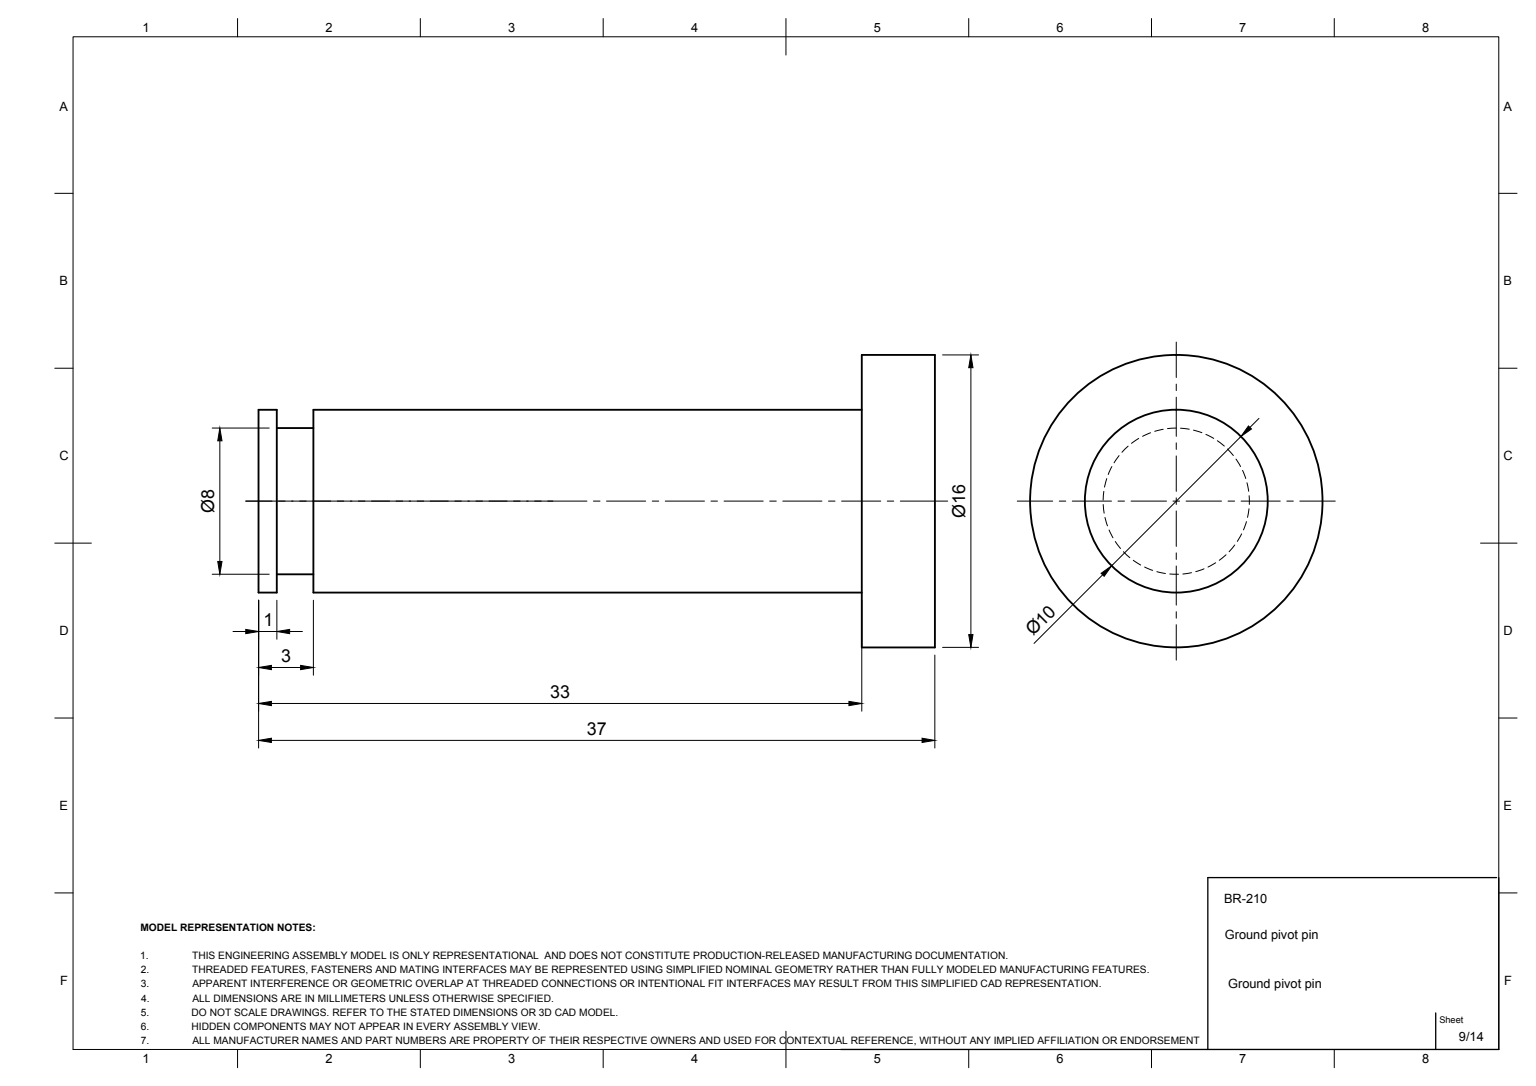
ISO-10303-21;
HEADER;
/* Generated by software containing ST-Developer
 * from STEP Tools, Inc. (www.steptools.com) 
 */

FILE_DESCRIPTION(
/* description */ ('Independent 1:2 reduction pantograph. 120 mm parallelogram sides; fix
ed fulcrum on the extension of a 240 mm link. Drawing point halfway al
ong its link, so its XY displacement is one half of the tracing point.
 Replaceable pivot bushes and retained pins. Calibration and productio
n accuracy unassigned.'),
/* implementation_level */ '2;1');

FILE_NAME(
/* name */ 'Ground pivot pin.step',
/* time_stamp */ '2026-11-07T22:11:57-08:00',
/* author */ (''),
/* organization */ (''),
/* preprocessor_version */ 'ST-DEVELOPER v20.2',
/* originating_system */ 'Autodesk Translation Framework v15.17.0.0',
/* authorisation */ '');

FILE_SCHEMA (('AUTOMOTIVE_DESIGN { 1 0 10303 214 3 1 1 }'));
ENDSEC;

DATA;
#10=MECHANICAL_DESIGN_GEOMETRIC_PRESENTATION_REPRESENTATION('',(#190),#2926);
#164=SHAPE_REPRESENTATION_RELATIONSHIP('SRR','None',#3001,#177);
#177=ADVANCED_BREP_SHAPE_REPRESENTATION('',(#203),#2917);
#190=STYLED_ITEM('',(#3075),#203);
#203=MANIFOLD_SOLID_BREP('Body1',#1545);
#236=FACE_BOUND('',#456,.T.);
#237=FACE_BOUND('',#458,.T.);
#238=FACE_BOUND('',#461,.T.);
#274=PLANE('',#1774);
#275=PLANE('',#1776);
#276=PLANE('',#1780);
#277=PLANE('',#1785);
#278=PLANE('',#1787);
#338=FACE_OUTER_BOUND('',#454,.T.);
#339=FACE_OUTER_BOUND('',#455,.T.);
#340=FACE_OUTER_BOUND('',#457,.T.);
#341=FACE_OUTER_BOUND('',#459,.T.);
#342=FACE_OUTER_BOUND('',#460,.T.);
#343=FACE_OUTER_BOUND('',#462,.T.);
#344=FACE_OUTER_BOUND('',#463,.T.);
#345=FACE_OUTER_BOUND('',#464,.T.);
#346=FACE_OUTER_BOUND('',#465,.T.);
#454=EDGE_LOOP('',(#1217,#1218,#1219,#1220));
#455=EDGE_LOOP('',(#1221));
#456=EDGE_LOOP('',(#1222));
#457=EDGE_LOOP('',(#1223));
#458=EDGE_LOOP('',(#1224));
#459=EDGE_LOOP('',(#1225,#1226,#1227,#1228));
#460=EDGE_LOOP('',(#1229));
#461=EDGE_LOOP('',(#1230));
#462=EDGE_LOOP('',(#1231,#1232,#1233,#1234));
#463=EDGE_LOOP('',(#1235));
#464=EDGE_LOOP('',(#1236,#1237,#1238,#1239));
#465=EDGE_LOOP('',(#1240));
#576=LINE('',#2640,#657);
#577=LINE('',#2651,#658);
#578=LINE('',#2659,#659);
#579=LINE('',#2663,#660);
#657=VECTOR('',#2120,4.);
#658=VECTOR('',#2135,5.);
#659=VECTOR('',#2144,8.);
#660=VECTOR('',#2151,5.);
#731=CIRCLE('',#1772,4.);
#732=CIRCLE('',#1773,4.);
#733=CIRCLE('',#1775,5.);
#734=CIRCLE('',#1777,5.);
#735=CIRCLE('',#1779,5.);
#736=CIRCLE('',#1781,8.);
#737=CIRCLE('',#1782,5.);
#738=CIRCLE('',#1784,8.);
#835=VERTEX_POINT('',#2637);
#836=VERTEX_POINT('',#2639);
#837=VERTEX_POINT('',#2643);
#838=VERTEX_POINT('',#2646);
#839=VERTEX_POINT('',#2649);
#840=VERTEX_POINT('',#2653);
#841=VERTEX_POINT('',#2655);
#842=VERTEX_POINT('',#2658);
#973=EDGE_CURVE('',#835,#835,#731,.T.);
#974=EDGE_CURVE('',#835,#836,#576,.T.);
#975=EDGE_CURVE('',#836,#836,#732,.T.);
#976=EDGE_CURVE('',#837,#837,#733,.T.);
#977=EDGE_CURVE('',#838,#838,#734,.T.);
#978=EDGE_CURVE('',#839,#839,#735,.T.);
#979=EDGE_CURVE('',#839,#838,#577,.T.);
#980=EDGE_CURVE('',#840,#840,#736,.T.);
#981=EDGE_CURVE('',#841,#841,#737,.T.);
#982=EDGE_CURVE('',#840,#842,#578,.T.);
#983=EDGE_CURVE('',#842,#842,#738,.T.);
#984=EDGE_CURVE('',#837,#841,#579,.T.);
#1217=ORIENTED_EDGE('',*,*,#973,.T.);
#1218=ORIENTED_EDGE('',*,*,#974,.T.);
#1219=ORIENTED_EDGE('',*,*,#975,.F.);
#1220=ORIENTED_EDGE('',*,*,#974,.F.);
#1221=ORIENTED_EDGE('',*,*,#976,.F.);
#1222=ORIENTED_EDGE('',*,*,#973,.F.);
#1223=ORIENTED_EDGE('',*,*,#977,.F.);
#1224=ORIENTED_EDGE('',*,*,#975,.T.);
#1225=ORIENTED_EDGE('',*,*,#978,.F.);
#1226=ORIENTED_EDGE('',*,*,#979,.T.);
#1227=ORIENTED_EDGE('',*,*,#977,.T.);
#1228=ORIENTED_EDGE('',*,*,#979,.F.);
#1229=ORIENTED_EDGE('',*,*,#980,.T.);
#1230=ORIENTED_EDGE('',*,*,#981,.F.);
#1231=ORIENTED_EDGE('',*,*,#980,.F.);
#1232=ORIENTED_EDGE('',*,*,#982,.T.);
#1233=ORIENTED_EDGE('',*,*,#983,.T.);
#1234=ORIENTED_EDGE('',*,*,#982,.F.);
#1235=ORIENTED_EDGE('',*,*,#983,.F.);
#1236=ORIENTED_EDGE('',*,*,#976,.T.);
#1237=ORIENTED_EDGE('',*,*,#984,.T.);
#1238=ORIENTED_EDGE('',*,*,#981,.T.);
#1239=ORIENTED_EDGE('',*,*,#984,.F.);
#1240=ORIENTED_EDGE('',*,*,#978,.T.);
#1422=CYLINDRICAL_SURFACE('',#1771,4.);
#1423=CYLINDRICAL_SURFACE('',#1778,5.);
#1424=CYLINDRICAL_SURFACE('',#1783,8.);
#1425=CYLINDRICAL_SURFACE('',#1786,5.);
#1482=ADVANCED_FACE('',(#338),#1422,.T.);
#1483=ADVANCED_FACE('',(#339,#236),#274,.F.);
#1484=ADVANCED_FACE('',(#340,#237),#275,.F.);
#1485=ADVANCED_FACE('',(#341),#1423,.T.);
#1486=ADVANCED_FACE('',(#342,#238),#276,.T.);
#1487=ADVANCED_FACE('',(#343),#1424,.T.);
#1488=ADVANCED_FACE('',(#344),#277,.F.);
#1489=ADVANCED_FACE('',(#345),#1425,.T.);
#1490=ADVANCED_FACE('',(#346),#278,.T.);
#1545=CLOSED_SHELL('',(#1482,#1483,#1484,#1485,#1486,#1487,#1488,#1489,
#1490));
#1770=AXIS2_PLACEMENT_3D('',#2635,#2114,#2115);
#1771=AXIS2_PLACEMENT_3D('',#2636,#2116,#2117);
#1772=AXIS2_PLACEMENT_3D('',#2638,#2118,#2119);
#1773=AXIS2_PLACEMENT_3D('',#2641,#2121,#2122);
#1774=AXIS2_PLACEMENT_3D('',#2642,#2123,#2124);
#1775=AXIS2_PLACEMENT_3D('',#2644,#2125,#2126);
#1776=AXIS2_PLACEMENT_3D('',#2645,#2127,#2128);
#1777=AXIS2_PLACEMENT_3D('',#2647,#2129,#2130);
#1778=AXIS2_PLACEMENT_3D('',#2648,#2131,#2132);
#1779=AXIS2_PLACEMENT_3D('',#2650,#2133,#2134);
#1780=AXIS2_PLACEMENT_3D('',#2652,#2136,#2137);
#1781=AXIS2_PLACEMENT_3D('',#2654,#2138,#2139);
#1782=AXIS2_PLACEMENT_3D('',#2656,#2140,#2141);
#1783=AXIS2_PLACEMENT_3D('',#2657,#2142,#2143);
#1784=AXIS2_PLACEMENT_3D('',#2660,#2145,#2146);
#1785=AXIS2_PLACEMENT_3D('',#2661,#2147,#2148);
#1786=AXIS2_PLACEMENT_3D('',#2662,#2149,#2150);
#1787=AXIS2_PLACEMENT_3D('',#2664,#2152,#2153);
#2114=DIRECTION('axis',(0.,0.,1.));
#2115=DIRECTION('refdir',(1.,0.,0.));
#2116=DIRECTION('center_axis',(0.,0.,1.));
#2117=DIRECTION('ref_axis',(1.,0.,0.));
#2118=DIRECTION('center_axis',(0.,0.,1.));
#2119=DIRECTION('ref_axis',(1.,0.,0.));
#2120=DIRECTION('',(0.,0.,1.));
#2121=DIRECTION('center_axis',(0.,0.,1.));
#2122=DIRECTION('ref_axis',(1.,0.,0.));
#2123=DIRECTION('center_axis',(0.,0.,-1.));
#2124=DIRECTION('ref_axis',(-1.,0.,0.));
#2125=DIRECTION('center_axis',(0.,0.,-1.));
#2126=DIRECTION('ref_axis',(1.,0.,0.));
#2127=DIRECTION('center_axis',(0.,0.,1.));
#2128=DIRECTION('ref_axis',(1.,0.,0.));
#2129=DIRECTION('center_axis',(0.,0.,1.));
#2130=DIRECTION('ref_axis',(1.,0.,0.));
#2131=DIRECTION('center_axis',(0.,0.,1.));
#2132=DIRECTION('ref_axis',(1.,0.,0.));
#2133=DIRECTION('center_axis',(0.,0.,1.));
#2134=DIRECTION('ref_axis',(1.,0.,0.));
#2135=DIRECTION('',(0.,0.,-1.));
#2136=DIRECTION('center_axis',(0.,0.,1.));
#2137=DIRECTION('ref_axis',(1.,0.,0.));
#2138=DIRECTION('center_axis',(0.,0.,1.));
#2139=DIRECTION('ref_axis',(1.,0.,0.));
#2140=DIRECTION('center_axis',(0.,0.,1.));
#2141=DIRECTION('ref_axis',(1.,0.,0.));
#2142=DIRECTION('center_axis',(0.,0.,1.));
#2143=DIRECTION('ref_axis',(1.,0.,0.));
#2144=DIRECTION('',(0.,0.,-1.));
#2145=DIRECTION('center_axis',(0.,0.,1.));
#2146=DIRECTION('ref_axis',(1.,0.,0.));
#2147=DIRECTION('center_axis',(0.,0.,1.));
#2148=DIRECTION('ref_axis',(1.,0.,0.));
#2149=DIRECTION('center_axis',(0.,0.,1.));
#2150=DIRECTION('ref_axis',(1.,0.,0.));
#2151=DIRECTION('',(0.,0.,-1.));
#2152=DIRECTION('center_axis',(0.,0.,1.));
#2153=DIRECTION('ref_axis',(1.,0.,0.));
#2635=CARTESIAN_POINT('',(0.,0.,0.));
#2636=CARTESIAN_POINT('Origin',(0.,0.,31.));
#2637=CARTESIAN_POINT('',(-4.,-4.89858719658941E-16,30.));
#2638=CARTESIAN_POINT('Origin',(0.,0.,30.));
#2639=CARTESIAN_POINT('',(-4.,-4.89858719658941E-16,32.));
#2640=CARTESIAN_POINT('',(-4.,-4.89858719658941E-16,31.));
#2641=CARTESIAN_POINT('Origin',(0.,0.,32.));
#2642=CARTESIAN_POINT('Origin',(8.,0.,30.));
#2643=CARTESIAN_POINT('',(-5.,6.12323399573677E-16,30.));
#2644=CARTESIAN_POINT('Origin',(0.,0.,30.));
#2645=CARTESIAN_POINT('Origin',(4.,0.,32.));
#2646=CARTESIAN_POINT('',(-5.,-6.12323399573677E-16,32.));
#2647=CARTESIAN_POINT('Origin',(0.,0.,32.));
#2648=CARTESIAN_POINT('Origin',(0.,0.,0.));
#2649=CARTESIAN_POINT('',(-5.,-6.12323399573677E-16,33.));
#2650=CARTESIAN_POINT('Origin',(0.,0.,33.));
#2651=CARTESIAN_POINT('',(-5.,-6.12323399573677E-16,0.));
#2652=CARTESIAN_POINT('Origin',(0.,0.,0.));
#2653=CARTESIAN_POINT('',(-8.,-9.79717439317883E-16,0.));
#2654=CARTESIAN_POINT('Origin',(0.,0.,0.));
#2655=CARTESIAN_POINT('',(-5.,-6.12323399573677E-16,0.));
#2656=CARTESIAN_POINT('Origin',(0.,0.,0.));
#2657=CARTESIAN_POINT('Origin',(0.,0.,-4.));
#2658=CARTESIAN_POINT('',(-8.,-9.79717439317883E-16,-4.));
#2659=CARTESIAN_POINT('',(-8.,-9.79717439317883E-16,-4.));
#2660=CARTESIAN_POINT('Origin',(0.,0.,-4.));
#2661=CARTESIAN_POINT('Origin',(0.,0.,-4.));
#2662=CARTESIAN_POINT('Origin',(0.,0.,0.));
#2663=CARTESIAN_POINT('',(-5.,-6.12323399573677E-16,0.));
#2664=CARTESIAN_POINT('Origin',(0.,0.,33.));
#2902=UNCERTAINTY_MEASURE_WITH_UNIT(LENGTH_MEASURE(0.01),#2927,
'DISTANCE_ACCURACY_VALUE',
'Maximum model space distance between geometric entities at asserted c
onnectivities');
#2911=UNCERTAINTY_MEASURE_WITH_UNIT(LENGTH_MEASURE(0.01),#2927,
'DISTANCE_ACCURACY_VALUE',
'Maximum model space distance between geometric entities at asserted c
onnectivities');
#2917=(
GEOMETRIC_REPRESENTATION_CONTEXT(3)
GLOBAL_UNCERTAINTY_ASSIGNED_CONTEXT((#2902))
GLOBAL_UNIT_ASSIGNED_CONTEXT((#2927,#2929,#2930))
REPRESENTATION_CONTEXT('','3D')
);
#2926=(
GEOMETRIC_REPRESENTATION_CONTEXT(3)
GLOBAL_UNCERTAINTY_ASSIGNED_CONTEXT((#2911))
GLOBAL_UNIT_ASSIGNED_CONTEXT((#2927,#2929,#2930))
REPRESENTATION_CONTEXT('','3D')
);
#2927=(
LENGTH_UNIT()
NAMED_UNIT(*)
SI_UNIT(.MILLI.,.METRE.)
);
#2929=(
NAMED_UNIT(*)
PLANE_ANGLE_UNIT()
SI_UNIT($,.RADIAN.)
);
#2930=(
NAMED_UNIT(*)
SI_UNIT($,.STERADIAN.)
SOLID_ANGLE_UNIT()
);
#2936=SHAPE_DEFINITION_REPRESENTATION(#2950,#3001);
#2950=PRODUCT_DEFINITION_SHAPE('',$,#3016);
#3001=SHAPE_REPRESENTATION('',(#1770),#2917);
#3010=PRODUCT_DEFINITION_CONTEXT('part definition',#3054,'design');
#3016=PRODUCT_DEFINITION('Ground pivot pin','Ground pivot pin',#3030,#3010);
#3030=PRODUCT_DEFINITION_FORMATION('',$,#3061);
#3054=APPLICATION_CONTEXT(
'Core Data for Automotive Mechanical Design Process');
#3055=PRODUCT_CONTEXT('part definition',#3054,'mechanical');
#3061=PRODUCT('Ground pivot pin','Ground pivot pin',$,(#3055));
#3075=PRESENTATION_STYLE_ASSIGNMENT((#3087));
#3087=SURFACE_STYLE_USAGE(.BOTH.,#3099);
#3099=SURFACE_SIDE_STYLE('',(#3111));
#3111=SURFACE_STYLE_FILL_AREA(#3123);
#3123=FILL_AREA_STYLE('Pivot gray',(#3135));
#3135=FILL_AREA_STYLE_COLOUR('Pivot gray',#3147);
#3147=COLOUR_RGB('Pivot gray',0.407843137254902,0.447058823529412,0.498039215686275);
ENDSEC;
END-ISO-10303-21;
